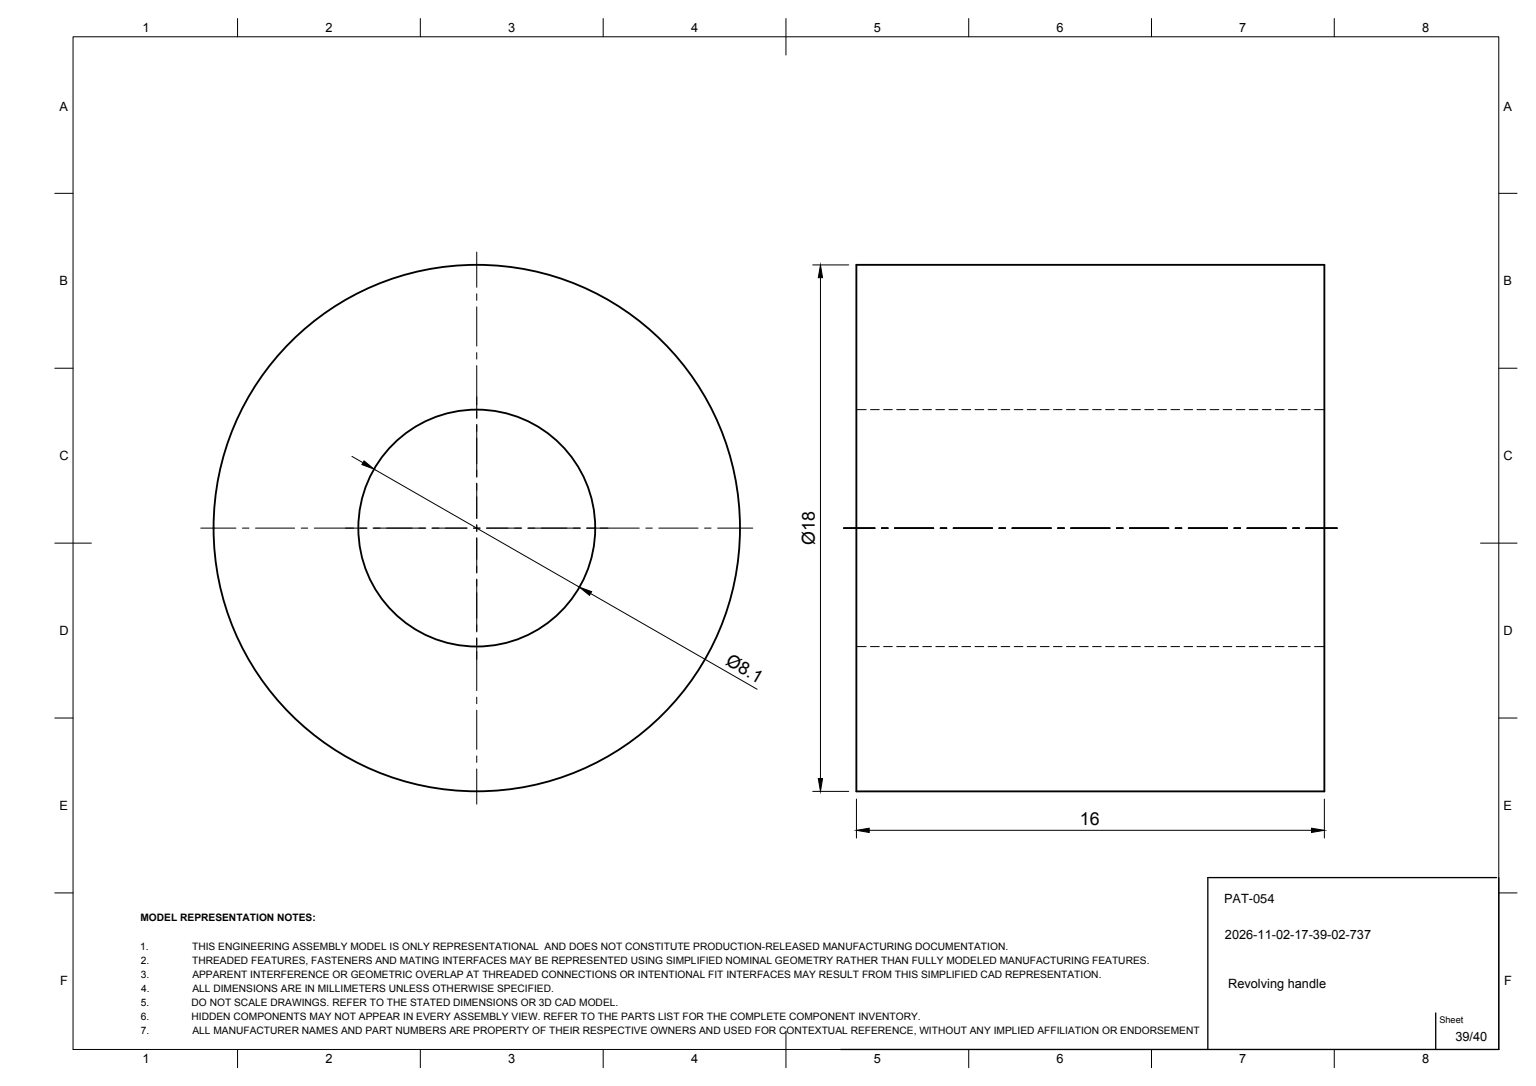
ISO-10303-21;
HEADER;
/* Generated by software containing ST-Developer
 * from STEP Tools, Inc. (www.steptools.com) 
 */

FILE_DESCRIPTION(
/* description */ ('PAT-054'),
/* implementation_level */ '2;1');

FILE_NAME(
/* name */ 'Revolving handle.step',
/* time_stamp */ '2026-10-29T16:38:13-07:00',
/* author */ (''),
/* organization */ (''),
/* preprocessor_version */ 'ST-DEVELOPER v20.2',
/* originating_system */ 'Autodesk Translation Framework v15.17.0.0',
/* authorisation */ '');

FILE_SCHEMA (('AUTOMOTIVE_DESIGN { 1 0 10303 214 3 1 1 }'));
ENDSEC;

DATA;
#10=MECHANICAL_DESIGN_GEOMETRIC_PRESENTATION_REPRESENTATION('',(#953),#33981);
#850=SHAPE_REPRESENTATION_RELATIONSHIP('SRR','None',#34228,#894);
#894=ADVANCED_BREP_SHAPE_REPRESENTATION('',(#1008),#33976);
#953=STYLED_ITEM('',(#34510),#1008);
#1008=MANIFOLD_SOLID_BREP('Body1',#13068);
#1222=FACE_BOUND('',#3187,.T.);
#1223=FACE_BOUND('',#3189,.T.);
#1541=PLANE('',#14764);
#1542=PLANE('',#14765);
#2251=FACE_OUTER_BOUND('',#3184,.T.);
#2252=FACE_OUTER_BOUND('',#3185,.T.);
#2253=FACE_OUTER_BOUND('',#3186,.T.);
#2254=FACE_OUTER_BOUND('',#3188,.T.);
#3184=EDGE_LOOP('',(#11793,#11794,#11795,#11796));
#3185=EDGE_LOOP('',(#11797,#11798,#11799,#11800));
#3186=EDGE_LOOP('',(#11801));
#3187=EDGE_LOOP('',(#11802));
#3188=EDGE_LOOP('',(#11803));
#3189=EDGE_LOOP('',(#11804));
#4098=LINE('',#33617,#5032);
#4099=LINE('',#33623,#5033);
#5032=VECTOR('',#18153,0.405);
#5033=VECTOR('',#18160,0.9);
#5550=CIRCLE('',#14759,0.405);
#5551=CIRCLE('',#14760,0.405);
#5552=CIRCLE('',#14762,0.9);
#5553=CIRCLE('',#14763,0.9);
#6684=VERTEX_POINT('',#33614);
#6685=VERTEX_POINT('',#33616);
#6686=VERTEX_POINT('',#33620);
#6687=VERTEX_POINT('',#33622);
#8396=EDGE_CURVE('',#6684,#6684,#5550,.T.);
#8397=EDGE_CURVE('',#6684,#6685,#4098,.T.);
#8398=EDGE_CURVE('',#6685,#6685,#5551,.T.);
#8399=EDGE_CURVE('',#6686,#6686,#5552,.T.);
#8400=EDGE_CURVE('',#6686,#6687,#4099,.T.);
#8401=EDGE_CURVE('',#6687,#6687,#5553,.T.);
#11793=ORIENTED_EDGE('',*,*,#8396,.F.);
#11794=ORIENTED_EDGE('',*,*,#8397,.T.);
#11795=ORIENTED_EDGE('',*,*,#8398,.T.);
#11796=ORIENTED_EDGE('',*,*,#8397,.F.);
#11797=ORIENTED_EDGE('',*,*,#8399,.F.);
#11798=ORIENTED_EDGE('',*,*,#8400,.T.);
#11799=ORIENTED_EDGE('',*,*,#8401,.T.);
#11800=ORIENTED_EDGE('',*,*,#8400,.F.);
#11801=ORIENTED_EDGE('',*,*,#8399,.T.);
#11802=ORIENTED_EDGE('',*,*,#8396,.T.);
#11803=ORIENTED_EDGE('',*,*,#8401,.F.);
#11804=ORIENTED_EDGE('',*,*,#8398,.F.);
#12280=CYLINDRICAL_SURFACE('',#14758,0.405);
#12281=CYLINDRICAL_SURFACE('',#14761,0.9);
#12963=ADVANCED_FACE('',(#2251),#12280,.F.);
#12964=ADVANCED_FACE('',(#2252),#12281,.T.);
#12965=ADVANCED_FACE('',(#2253,#1222),#1541,.T.);
#12966=ADVANCED_FACE('',(#2254,#1223),#1542,.F.);
#13068=CLOSED_SHELL('',(#12963,#12964,#12965,#12966));
#14757=AXIS2_PLACEMENT_3D('',#33612,#18147,#18148);
#14758=AXIS2_PLACEMENT_3D('',#33613,#18149,#18150);
#14759=AXIS2_PLACEMENT_3D('',#33615,#18151,#18152);
#14760=AXIS2_PLACEMENT_3D('',#33618,#18154,#18155);
#14761=AXIS2_PLACEMENT_3D('',#33619,#18156,#18157);
#14762=AXIS2_PLACEMENT_3D('',#33621,#18158,#18159);
#14763=AXIS2_PLACEMENT_3D('',#33624,#18161,#18162);
#14764=AXIS2_PLACEMENT_3D('',#33625,#18163,#18164);
#14765=AXIS2_PLACEMENT_3D('',#33626,#18165,#18166);
#18147=DIRECTION('axis',(0.,0.,1.));
#18148=DIRECTION('refdir',(1.,0.,0.));
#18149=DIRECTION('center_axis',(1.,0.,0.));
#18150=DIRECTION('ref_axis',(0.,0.,-1.));
#18151=DIRECTION('center_axis',(-1.,0.,0.));
#18152=DIRECTION('ref_axis',(0.,0.,-1.));
#18153=DIRECTION('',(-1.,0.,0.));
#18154=DIRECTION('center_axis',(-1.,0.,0.));
#18155=DIRECTION('ref_axis',(0.,0.,-1.));
#18156=DIRECTION('center_axis',(1.,0.,0.));
#18157=DIRECTION('ref_axis',(0.,0.,-1.));
#18158=DIRECTION('center_axis',(1.,0.,0.));
#18159=DIRECTION('ref_axis',(0.,0.,-1.));
#18160=DIRECTION('',(-1.,0.,0.));
#18161=DIRECTION('center_axis',(1.,0.,0.));
#18162=DIRECTION('ref_axis',(0.,0.,-1.));
#18163=DIRECTION('center_axis',(1.,0.,0.));
#18164=DIRECTION('ref_axis',(0.,0.,-1.));
#18165=DIRECTION('center_axis',(1.,0.,0.));
#18166=DIRECTION('ref_axis',(0.,0.,-1.));
#33612=CARTESIAN_POINT('',(0.,0.,0.));
#33613=CARTESIAN_POINT('Origin',(29.4,0.,6.5));
#33614=CARTESIAN_POINT('',(31.,-4.95981953654678E-17,6.905));
#33615=CARTESIAN_POINT('Origin',(31.,0.,6.5));
#33616=CARTESIAN_POINT('',(29.4,-4.95981953654678E-17,6.905));
#33617=CARTESIAN_POINT('',(29.4,-4.95981953654678E-17,6.905));
#33618=CARTESIAN_POINT('Origin',(29.4,0.,6.5));
#33619=CARTESIAN_POINT('Origin',(29.4,0.,6.5));
#33620=CARTESIAN_POINT('',(31.,-1.10218211923262E-16,7.4));
#33621=CARTESIAN_POINT('Origin',(31.,0.,6.5));
#33622=CARTESIAN_POINT('',(29.4,-1.10218211923262E-16,7.4));
#33623=CARTESIAN_POINT('',(29.4,-1.10218211923262E-16,7.4));
#33624=CARTESIAN_POINT('Origin',(29.4,0.,6.5));
#33625=CARTESIAN_POINT('Origin',(31.,0.,6.5));
#33626=CARTESIAN_POINT('Origin',(29.4,0.,6.5));
#33924=UNCERTAINTY_MEASURE_WITH_UNIT(LENGTH_MEASURE(0.001),#33982,
'DISTANCE_ACCURACY_VALUE',
'Maximum model space distance between geometric entities at asserted c
onnectivities');
#33929=UNCERTAINTY_MEASURE_WITH_UNIT(LENGTH_MEASURE(0.001),#33982,
'DISTANCE_ACCURACY_VALUE',
'Maximum model space distance between geometric entities at asserted c
onnectivities');
#33976=(
GEOMETRIC_REPRESENTATION_CONTEXT(3)
GLOBAL_UNCERTAINTY_ASSIGNED_CONTEXT((#33924))
GLOBAL_UNIT_ASSIGNED_CONTEXT((#33982,#33984,#33985))
REPRESENTATION_CONTEXT('','3D')
);
#33981=(
GEOMETRIC_REPRESENTATION_CONTEXT(3)
GLOBAL_UNCERTAINTY_ASSIGNED_CONTEXT((#33929))
GLOBAL_UNIT_ASSIGNED_CONTEXT((#33982,#33984,#33985))
REPRESENTATION_CONTEXT('','3D')
);
#33982=(
LENGTH_UNIT()
NAMED_UNIT(*)
SI_UNIT(.CENTI.,.METRE.)
);
#33984=(
NAMED_UNIT(*)
PLANE_ANGLE_UNIT()
SI_UNIT($,.RADIAN.)
);
#33985=(
NAMED_UNIT(*)
SI_UNIT($,.STERADIAN.)
SOLID_ANGLE_UNIT()
);
#34032=SHAPE_DEFINITION_REPRESENTATION(#34116,#34228);
#34116=PRODUCT_DEFINITION_SHAPE('',$,#34280);
#34228=SHAPE_REPRESENTATION('',(#14757),#33976);
#34233=PRODUCT_DEFINITION_CONTEXT('part definition',#34388,'design');
#34280=PRODUCT_DEFINITION('Revolving handle','Revolving handle',#34331,
#34233);
#34331=PRODUCT_DEFINITION_FORMATION('',$,#34436);
#34388=APPLICATION_CONTEXT(
'Core Data for Automotive Mechanical Design Process');
#34389=PRODUCT_CONTEXT('part definition',#34388,'mechanical');
#34436=PRODUCT('Revolving handle','Revolving handle','Revolving handle',
(#34389));
#34504=COLOUR_RGB('Sky Blue',0.24,0.69,0.87);
#34505=FILL_AREA_STYLE_COLOUR('',#34504);
#34506=FILL_AREA_STYLE('',(#34505));
#34507=SURFACE_STYLE_FILL_AREA(#34506);
#34508=SURFACE_SIDE_STYLE('',(#34507));
#34509=SURFACE_STYLE_USAGE(.BOTH.,#34508);
#34510=PRESENTATION_STYLE_ASSIGNMENT((#34509));
ENDSEC;
END-ISO-10303-21;
